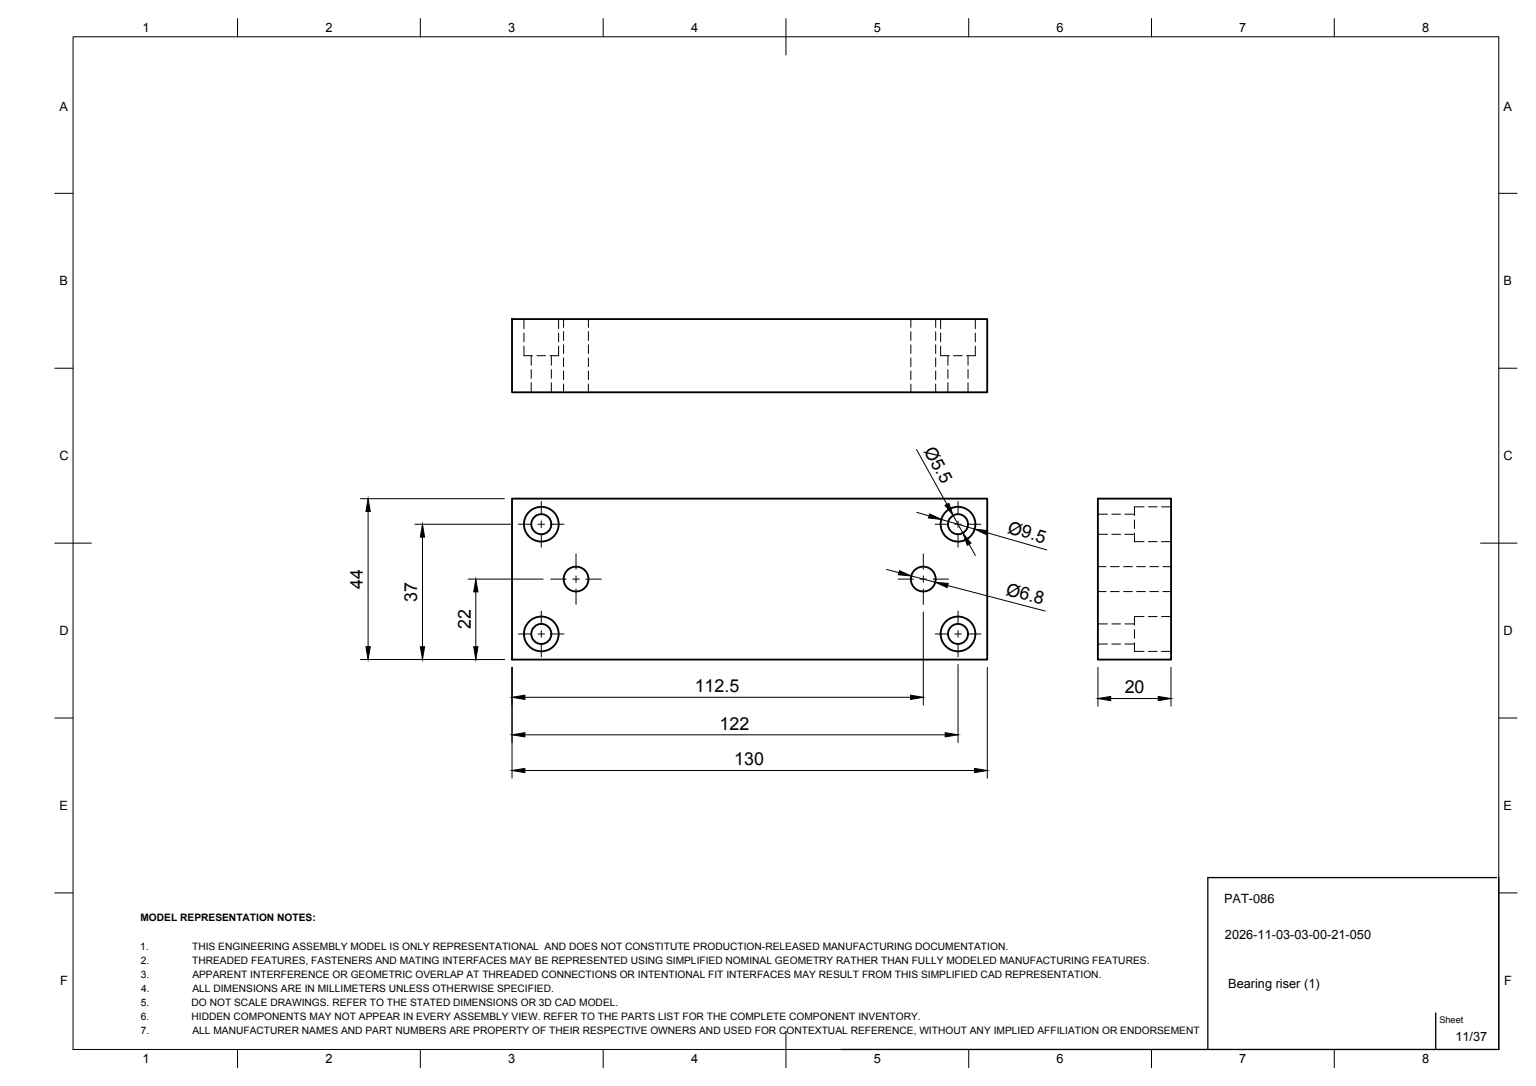
ISO-10303-21;
HEADER;
/* Generated by software containing ST-Developer
 * from STEP Tools, Inc. (www.steptools.com) 
 */

FILE_DESCRIPTION(
/* description */ ('Ratchet and pawl hand winch drum'),
/* implementation_level */ '2;1');

FILE_NAME(
/* name */ 'Bearing riser (1).step',
/* time_stamp */ '2026-10-27T12:42:58-07:00',
/* author */ (''),
/* organization */ (''),
/* preprocessor_version */ 'ST-DEVELOPER v20.2',
/* originating_system */ 'Autodesk Translation Framework v15.17.0.0',
/* authorisation */ '');

FILE_SCHEMA (('AUTOMOTIVE_DESIGN { 1 0 10303 214 3 1 1 }'));
ENDSEC;

DATA;
#10=MECHANICAL_DESIGN_GEOMETRIC_PRESENTATION_REPRESENTATION('',(#395),#11801);
#327=SHAPE_REPRESENTATION_RELATIONSHIP('SRR','None',#11953,#361);
#361=ADVANCED_BREP_SHAPE_REPRESENTATION('',(#430),#11770);
#395=STYLED_ITEM('',(#12213),#430);
#430=MANIFOLD_SOLID_BREP('Body1',#6272);
#496=FACE_BOUND('',#1294,.T.);
#497=FACE_BOUND('',#1297,.T.);
#498=FACE_BOUND('',#1302,.T.);
#499=FACE_BOUND('',#1305,.T.);
#500=FACE_BOUND('',#1315,.T.);
#501=FACE_BOUND('',#1316,.T.);
#502=FACE_BOUND('',#1317,.T.);
#503=FACE_BOUND('',#1318,.T.);
#504=FACE_BOUND('',#1319,.T.);
#505=FACE_BOUND('',#1320,.T.);
#506=FACE_BOUND('',#1322,.T.);
#507=FACE_BOUND('',#1323,.T.);
#508=FACE_BOUND('',#1324,.T.);
#509=FACE_BOUND('',#1325,.T.);
#510=FACE_BOUND('',#1326,.T.);
#511=FACE_BOUND('',#1327,.T.);
#633=PLANE('',#6795);
#634=PLANE('',#6800);
#635=PLANE('',#6809);
#636=PLANE('',#6814);
#637=PLANE('',#6826);
#638=PLANE('',#6827);
#639=PLANE('',#6828);
#640=PLANE('',#6829);
#641=PLANE('',#6830);
#642=PLANE('',#6831);
#896=FACE_OUTER_BOUND('',#1292,.T.);
#897=FACE_OUTER_BOUND('',#1293,.T.);
#898=FACE_OUTER_BOUND('',#1295,.T.);
#899=FACE_OUTER_BOUND('',#1296,.T.);
#900=FACE_OUTER_BOUND('',#1298,.T.);
#901=FACE_OUTER_BOUND('',#1299,.T.);
#902=FACE_OUTER_BOUND('',#1300,.T.);
#903=FACE_OUTER_BOUND('',#1301,.T.);
#904=FACE_OUTER_BOUND('',#1303,.T.);
#905=FACE_OUTER_BOUND('',#1304,.T.);
#906=FACE_OUTER_BOUND('',#1306,.T.);
#907=FACE_OUTER_BOUND('',#1307,.T.);
#908=FACE_OUTER_BOUND('',#1308,.T.);
#909=FACE_OUTER_BOUND('',#1309,.T.);
#910=FACE_OUTER_BOUND('',#1310,.T.);
#911=FACE_OUTER_BOUND('',#1311,.T.);
#912=FACE_OUTER_BOUND('',#1312,.T.);
#913=FACE_OUTER_BOUND('',#1313,.T.);
#914=FACE_OUTER_BOUND('',#1314,.T.);
#915=FACE_OUTER_BOUND('',#1321,.T.);
#1292=EDGE_LOOP('',(#4487,#4488,#4489,#4490));
#1293=EDGE_LOOP('',(#4491));
#1294=EDGE_LOOP('',(#4492));
#1295=EDGE_LOOP('',(#4493,#4494,#4495,#4496));
#1296=EDGE_LOOP('',(#4497));
#1297=EDGE_LOOP('',(#4498));
#1298=EDGE_LOOP('',(#4499,#4500,#4501,#4502));
#1299=EDGE_LOOP('',(#4503,#4504,#4505,#4506));
#1300=EDGE_LOOP('',(#4507,#4508,#4509,#4510));
#1301=EDGE_LOOP('',(#4511));
#1302=EDGE_LOOP('',(#4512));
#1303=EDGE_LOOP('',(#4513,#4514,#4515,#4516));
#1304=EDGE_LOOP('',(#4517));
#1305=EDGE_LOOP('',(#4518));
#1306=EDGE_LOOP('',(#4519,#4520,#4521,#4522));
#1307=EDGE_LOOP('',(#4523,#4524,#4525,#4526));
#1308=EDGE_LOOP('',(#4527,#4528,#4529,#4530));
#1309=EDGE_LOOP('',(#4531,#4532,#4533,#4534));
#1310=EDGE_LOOP('',(#4535,#4536,#4537,#4538));
#1311=EDGE_LOOP('',(#4539,#4540,#4541,#4542));
#1312=EDGE_LOOP('',(#4543,#4544,#4545,#4546));
#1313=EDGE_LOOP('',(#4547,#4548,#4549,#4550));
#1314=EDGE_LOOP('',(#4551,#4552,#4553,#4554));
#1315=EDGE_LOOP('',(#4555));
#1316=EDGE_LOOP('',(#4556));
#1317=EDGE_LOOP('',(#4557));
#1318=EDGE_LOOP('',(#4558));
#1319=EDGE_LOOP('',(#4559));
#1320=EDGE_LOOP('',(#4560));
#1321=EDGE_LOOP('',(#4561,#4562,#4563,#4564));
#1322=EDGE_LOOP('',(#4565));
#1323=EDGE_LOOP('',(#4566));
#1324=EDGE_LOOP('',(#4567));
#1325=EDGE_LOOP('',(#4568));
#1326=EDGE_LOOP('',(#4569));
#1327=EDGE_LOOP('',(#4570));
#1769=LINE('',#9496,#2280);
#1770=LINE('',#9505,#2281);
#1771=LINE('',#9513,#2282);
#1772=LINE('',#9517,#2283);
#1773=LINE('',#9522,#2284);
#1774=LINE('',#9531,#2285);
#1775=LINE('',#9539,#2286);
#1776=LINE('',#9543,#2287);
#1777=LINE('',#9548,#2288);
#1778=LINE('',#9554,#2289);
#1779=LINE('',#9559,#2290);
#1780=LINE('',#9561,#2291);
#1781=LINE('',#9563,#2292);
#1782=LINE('',#9564,#2293);
#1783=LINE('',#9567,#2294);
#1784=LINE('',#9569,#2295);
#1785=LINE('',#9570,#2296);
#1786=LINE('',#9573,#2297);
#1787=LINE('',#9575,#2298);
#1788=LINE('',#9576,#2299);
#1789=LINE('',#9578,#2300);
#1790=LINE('',#9579,#2301);
#2280=VECTOR('',#7660,0.475);
#2281=VECTOR('',#7671,0.475);
#2282=VECTOR('',#7682,0.275);
#2283=VECTOR('',#7687,0.275);
#2284=VECTOR('',#7692,0.475);
#2285=VECTOR('',#7703,0.475);
#2286=VECTOR('',#7714,0.275);
#2287=VECTOR('',#7719,0.275);
#2288=VECTOR('',#7724,0.34);
#2289=VECTOR('',#7731,0.34);
#2290=VECTOR('',#7736,1.);
#2291=VECTOR('',#7737,1.);
#2292=VECTOR('',#7738,1.);
#2293=VECTOR('',#7739,1.);
#2294=VECTOR('',#7742,1.);
#2295=VECTOR('',#7743,1.);
#2296=VECTOR('',#7744,1.);
#2297=VECTOR('',#7747,1.);
#2298=VECTOR('',#7748,1.);
#2299=VECTOR('',#7749,1.);
#2300=VECTOR('',#7752,1.);
#2301=VECTOR('',#7753,1.);
#2767=CIRCLE('',#6793,0.475);
#2768=CIRCLE('',#6794,0.475);
#2769=CIRCLE('',#6796,0.275);
#2770=CIRCLE('',#6798,0.475);
#2771=CIRCLE('',#6799,0.475);
#2772=CIRCLE('',#6801,0.275);
#2773=CIRCLE('',#6803,0.275);
#2774=CIRCLE('',#6805,0.275);
#2775=CIRCLE('',#6807,0.475);
#2776=CIRCLE('',#6808,0.475);
#2777=CIRCLE('',#6810,0.275);
#2778=CIRCLE('',#6812,0.475);
#2779=CIRCLE('',#6813,0.475);
#2780=CIRCLE('',#6815,0.275);
#2781=CIRCLE('',#6817,0.275);
#2782=CIRCLE('',#6819,0.275);
#2783=CIRCLE('',#6821,0.34);
#2784=CIRCLE('',#6822,0.34);
#2785=CIRCLE('',#6824,0.34);
#2786=CIRCLE('',#6825,0.34);
#3022=VERTEX_POINT('',#9493);
#3023=VERTEX_POINT('',#9495);
#3024=VERTEX_POINT('',#9499);
#3025=VERTEX_POINT('',#9502);
#3026=VERTEX_POINT('',#9504);
#3027=VERTEX_POINT('',#9508);
#3028=VERTEX_POINT('',#9511);
#3029=VERTEX_POINT('',#9515);
#3030=VERTEX_POINT('',#9519);
#3031=VERTEX_POINT('',#9521);
#3032=VERTEX_POINT('',#9525);
#3033=VERTEX_POINT('',#9528);
#3034=VERTEX_POINT('',#9530);
#3035=VERTEX_POINT('',#9534);
#3036=VERTEX_POINT('',#9537);
#3037=VERTEX_POINT('',#9541);
#3038=VERTEX_POINT('',#9545);
#3039=VERTEX_POINT('',#9547);
#3040=VERTEX_POINT('',#9551);
#3041=VERTEX_POINT('',#9553);
#3042=VERTEX_POINT('',#9557);
#3043=VERTEX_POINT('',#9558);
#3044=VERTEX_POINT('',#9560);
#3045=VERTEX_POINT('',#9562);
#3046=VERTEX_POINT('',#9566);
#3047=VERTEX_POINT('',#9568);
#3048=VERTEX_POINT('',#9572);
#3049=VERTEX_POINT('',#9574);
#3587=EDGE_CURVE('',#3022,#3022,#2767,.T.);
#3588=EDGE_CURVE('',#3022,#3023,#1769,.T.);
#3589=EDGE_CURVE('',#3023,#3023,#2768,.T.);
#3590=EDGE_CURVE('',#3024,#3024,#2769,.T.);
#3591=EDGE_CURVE('',#3025,#3025,#2770,.T.);
#3592=EDGE_CURVE('',#3025,#3026,#1770,.T.);
#3593=EDGE_CURVE('',#3026,#3026,#2771,.T.);
#3594=EDGE_CURVE('',#3027,#3027,#2772,.T.);
#3595=EDGE_CURVE('',#3028,#3028,#2773,.T.);
#3596=EDGE_CURVE('',#3028,#3024,#1771,.T.);
#3597=EDGE_CURVE('',#3029,#3029,#2774,.T.);
#3598=EDGE_CURVE('',#3029,#3027,#1772,.T.);
#3599=EDGE_CURVE('',#3030,#3030,#2775,.T.);
#3600=EDGE_CURVE('',#3030,#3031,#1773,.T.);
#3601=EDGE_CURVE('',#3031,#3031,#2776,.T.);
#3602=EDGE_CURVE('',#3032,#3032,#2777,.T.);
#3603=EDGE_CURVE('',#3033,#3033,#2778,.T.);
#3604=EDGE_CURVE('',#3033,#3034,#1774,.T.);
#3605=EDGE_CURVE('',#3034,#3034,#2779,.T.);
#3606=EDGE_CURVE('',#3035,#3035,#2780,.T.);
#3607=EDGE_CURVE('',#3036,#3036,#2781,.T.);
#3608=EDGE_CURVE('',#3036,#3032,#1775,.T.);
#3609=EDGE_CURVE('',#3037,#3037,#2782,.T.);
#3610=EDGE_CURVE('',#3037,#3035,#1776,.T.);
#3611=EDGE_CURVE('',#3038,#3038,#2783,.T.);
#3612=EDGE_CURVE('',#3038,#3039,#1777,.T.);
#3613=EDGE_CURVE('',#3039,#3039,#2784,.T.);
#3614=EDGE_CURVE('',#3040,#3040,#2785,.T.);
#3615=EDGE_CURVE('',#3040,#3041,#1778,.T.);
#3616=EDGE_CURVE('',#3041,#3041,#2786,.T.);
#3617=EDGE_CURVE('',#3042,#3043,#1779,.T.);
#3618=EDGE_CURVE('',#3043,#3044,#1780,.T.);
#3619=EDGE_CURVE('',#3045,#3044,#1781,.T.);
#3620=EDGE_CURVE('',#3042,#3045,#1782,.T.);
#3621=EDGE_CURVE('',#3046,#3042,#1783,.T.);
#3622=EDGE_CURVE('',#3047,#3045,#1784,.T.);
#3623=EDGE_CURVE('',#3046,#3047,#1785,.T.);
#3624=EDGE_CURVE('',#3048,#3046,#1786,.T.);
#3625=EDGE_CURVE('',#3049,#3047,#1787,.T.);
#3626=EDGE_CURVE('',#3048,#3049,#1788,.T.);
#3627=EDGE_CURVE('',#3043,#3048,#1789,.T.);
#3628=EDGE_CURVE('',#3044,#3049,#1790,.T.);
#4487=ORIENTED_EDGE('',*,*,#3587,.F.);
#4488=ORIENTED_EDGE('',*,*,#3588,.T.);
#4489=ORIENTED_EDGE('',*,*,#3589,.F.);
#4490=ORIENTED_EDGE('',*,*,#3588,.F.);
#4491=ORIENTED_EDGE('',*,*,#3587,.T.);
#4492=ORIENTED_EDGE('',*,*,#3590,.F.);
#4493=ORIENTED_EDGE('',*,*,#3591,.F.);
#4494=ORIENTED_EDGE('',*,*,#3592,.T.);
#4495=ORIENTED_EDGE('',*,*,#3593,.F.);
#4496=ORIENTED_EDGE('',*,*,#3592,.F.);
#4497=ORIENTED_EDGE('',*,*,#3591,.T.);
#4498=ORIENTED_EDGE('',*,*,#3594,.F.);
#4499=ORIENTED_EDGE('',*,*,#3595,.F.);
#4500=ORIENTED_EDGE('',*,*,#3596,.T.);
#4501=ORIENTED_EDGE('',*,*,#3590,.T.);
#4502=ORIENTED_EDGE('',*,*,#3596,.F.);
#4503=ORIENTED_EDGE('',*,*,#3597,.F.);
#4504=ORIENTED_EDGE('',*,*,#3598,.T.);
#4505=ORIENTED_EDGE('',*,*,#3594,.T.);
#4506=ORIENTED_EDGE('',*,*,#3598,.F.);
#4507=ORIENTED_EDGE('',*,*,#3599,.F.);
#4508=ORIENTED_EDGE('',*,*,#3600,.T.);
#4509=ORIENTED_EDGE('',*,*,#3601,.F.);
#4510=ORIENTED_EDGE('',*,*,#3600,.F.);
#4511=ORIENTED_EDGE('',*,*,#3599,.T.);
#4512=ORIENTED_EDGE('',*,*,#3602,.F.);
#4513=ORIENTED_EDGE('',*,*,#3603,.F.);
#4514=ORIENTED_EDGE('',*,*,#3604,.T.);
#4515=ORIENTED_EDGE('',*,*,#3605,.F.);
#4516=ORIENTED_EDGE('',*,*,#3604,.F.);
#4517=ORIENTED_EDGE('',*,*,#3603,.T.);
#4518=ORIENTED_EDGE('',*,*,#3606,.F.);
#4519=ORIENTED_EDGE('',*,*,#3607,.F.);
#4520=ORIENTED_EDGE('',*,*,#3608,.T.);
#4521=ORIENTED_EDGE('',*,*,#3602,.T.);
#4522=ORIENTED_EDGE('',*,*,#3608,.F.);
#4523=ORIENTED_EDGE('',*,*,#3609,.F.);
#4524=ORIENTED_EDGE('',*,*,#3610,.T.);
#4525=ORIENTED_EDGE('',*,*,#3606,.T.);
#4526=ORIENTED_EDGE('',*,*,#3610,.F.);
#4527=ORIENTED_EDGE('',*,*,#3611,.F.);
#4528=ORIENTED_EDGE('',*,*,#3612,.T.);
#4529=ORIENTED_EDGE('',*,*,#3613,.F.);
#4530=ORIENTED_EDGE('',*,*,#3612,.F.);
#4531=ORIENTED_EDGE('',*,*,#3614,.F.);
#4532=ORIENTED_EDGE('',*,*,#3615,.T.);
#4533=ORIENTED_EDGE('',*,*,#3616,.F.);
#4534=ORIENTED_EDGE('',*,*,#3615,.F.);
#4535=ORIENTED_EDGE('',*,*,#3617,.T.);
#4536=ORIENTED_EDGE('',*,*,#3618,.T.);
#4537=ORIENTED_EDGE('',*,*,#3619,.F.);
#4538=ORIENTED_EDGE('',*,*,#3620,.F.);
#4539=ORIENTED_EDGE('',*,*,#3621,.T.);
#4540=ORIENTED_EDGE('',*,*,#3620,.T.);
#4541=ORIENTED_EDGE('',*,*,#3622,.F.);
#4542=ORIENTED_EDGE('',*,*,#3623,.F.);
#4543=ORIENTED_EDGE('',*,*,#3624,.T.);
#4544=ORIENTED_EDGE('',*,*,#3623,.T.);
#4545=ORIENTED_EDGE('',*,*,#3625,.F.);
#4546=ORIENTED_EDGE('',*,*,#3626,.F.);
#4547=ORIENTED_EDGE('',*,*,#3627,.T.);
#4548=ORIENTED_EDGE('',*,*,#3626,.T.);
#4549=ORIENTED_EDGE('',*,*,#3628,.F.);
#4550=ORIENTED_EDGE('',*,*,#3618,.F.);
#4551=ORIENTED_EDGE('',*,*,#3628,.T.);
#4552=ORIENTED_EDGE('',*,*,#3625,.T.);
#4553=ORIENTED_EDGE('',*,*,#3622,.T.);
#4554=ORIENTED_EDGE('',*,*,#3619,.T.);
#4555=ORIENTED_EDGE('',*,*,#3616,.T.);
#4556=ORIENTED_EDGE('',*,*,#3613,.T.);
#4557=ORIENTED_EDGE('',*,*,#3605,.T.);
#4558=ORIENTED_EDGE('',*,*,#3601,.T.);
#4559=ORIENTED_EDGE('',*,*,#3593,.T.);
#4560=ORIENTED_EDGE('',*,*,#3589,.T.);
#4561=ORIENTED_EDGE('',*,*,#3627,.F.);
#4562=ORIENTED_EDGE('',*,*,#3617,.F.);
#4563=ORIENTED_EDGE('',*,*,#3621,.F.);
#4564=ORIENTED_EDGE('',*,*,#3624,.F.);
#4565=ORIENTED_EDGE('',*,*,#3595,.T.);
#4566=ORIENTED_EDGE('',*,*,#3597,.T.);
#4567=ORIENTED_EDGE('',*,*,#3607,.T.);
#4568=ORIENTED_EDGE('',*,*,#3609,.T.);
#4569=ORIENTED_EDGE('',*,*,#3611,.T.);
#4570=ORIENTED_EDGE('',*,*,#3614,.T.);
#5831=CYLINDRICAL_SURFACE('',#6792,0.475);
#5832=CYLINDRICAL_SURFACE('',#6797,0.475);
#5833=CYLINDRICAL_SURFACE('',#6802,0.275);
#5834=CYLINDRICAL_SURFACE('',#6804,0.275);
#5835=CYLINDRICAL_SURFACE('',#6806,0.475);
#5836=CYLINDRICAL_SURFACE('',#6811,0.475);
#5837=CYLINDRICAL_SURFACE('',#6816,0.275);
#5838=CYLINDRICAL_SURFACE('',#6818,0.275);
#5839=CYLINDRICAL_SURFACE('',#6820,0.34);
#5840=CYLINDRICAL_SURFACE('',#6823,0.34);
#5966=ADVANCED_FACE('',(#896),#5831,.F.);
#5967=ADVANCED_FACE('',(#897,#496),#633,.T.);
#5968=ADVANCED_FACE('',(#898),#5832,.F.);
#5969=ADVANCED_FACE('',(#899,#497),#634,.T.);
#5970=ADVANCED_FACE('',(#900),#5833,.F.);
#5971=ADVANCED_FACE('',(#901),#5834,.F.);
#5972=ADVANCED_FACE('',(#902),#5835,.F.);
#5973=ADVANCED_FACE('',(#903,#498),#635,.T.);
#5974=ADVANCED_FACE('',(#904),#5836,.F.);
#5975=ADVANCED_FACE('',(#905,#499),#636,.T.);
#5976=ADVANCED_FACE('',(#906),#5837,.F.);
#5977=ADVANCED_FACE('',(#907),#5838,.F.);
#5978=ADVANCED_FACE('',(#908),#5839,.F.);
#5979=ADVANCED_FACE('',(#909),#5840,.F.);
#5980=ADVANCED_FACE('',(#910),#637,.T.);
#5981=ADVANCED_FACE('',(#911),#638,.T.);
#5982=ADVANCED_FACE('',(#912),#639,.T.);
#5983=ADVANCED_FACE('',(#913),#640,.T.);
#5984=ADVANCED_FACE('',(#914,#500,#501,#502,#503,#504,#505),#641,.T.);
#5985=ADVANCED_FACE('',(#915,#506,#507,#508,#509,#510,#511),#642,.F.);
#6272=CLOSED_SHELL('',(#5966,#5967,#5968,#5969,#5970,#5971,#5972,#5973,
#5974,#5975,#5976,#5977,#5978,#5979,#5980,#5981,#5982,#5983,#5984,#5985));
#6791=AXIS2_PLACEMENT_3D('',#9491,#7654,#7655);
#6792=AXIS2_PLACEMENT_3D('',#9492,#7656,#7657);
#6793=AXIS2_PLACEMENT_3D('',#9494,#7658,#7659);
#6794=AXIS2_PLACEMENT_3D('',#9497,#7661,#7662);
#6795=AXIS2_PLACEMENT_3D('',#9498,#7663,#7664);
#6796=AXIS2_PLACEMENT_3D('',#9500,#7665,#7666);
#6797=AXIS2_PLACEMENT_3D('',#9501,#7667,#7668);
#6798=AXIS2_PLACEMENT_3D('',#9503,#7669,#7670);
#6799=AXIS2_PLACEMENT_3D('',#9506,#7672,#7673);
#6800=AXIS2_PLACEMENT_3D('',#9507,#7674,#7675);
#6801=AXIS2_PLACEMENT_3D('',#9509,#7676,#7677);
#6802=AXIS2_PLACEMENT_3D('',#9510,#7678,#7679);
#6803=AXIS2_PLACEMENT_3D('',#9512,#7680,#7681);
#6804=AXIS2_PLACEMENT_3D('',#9514,#7683,#7684);
#6805=AXIS2_PLACEMENT_3D('',#9516,#7685,#7686);
#6806=AXIS2_PLACEMENT_3D('',#9518,#7688,#7689);
#6807=AXIS2_PLACEMENT_3D('',#9520,#7690,#7691);
#6808=AXIS2_PLACEMENT_3D('',#9523,#7693,#7694);
#6809=AXIS2_PLACEMENT_3D('',#9524,#7695,#7696);
#6810=AXIS2_PLACEMENT_3D('',#9526,#7697,#7698);
#6811=AXIS2_PLACEMENT_3D('',#9527,#7699,#7700);
#6812=AXIS2_PLACEMENT_3D('',#9529,#7701,#7702);
#6813=AXIS2_PLACEMENT_3D('',#9532,#7704,#7705);
#6814=AXIS2_PLACEMENT_3D('',#9533,#7706,#7707);
#6815=AXIS2_PLACEMENT_3D('',#9535,#7708,#7709);
#6816=AXIS2_PLACEMENT_3D('',#9536,#7710,#7711);
#6817=AXIS2_PLACEMENT_3D('',#9538,#7712,#7713);
#6818=AXIS2_PLACEMENT_3D('',#9540,#7715,#7716);
#6819=AXIS2_PLACEMENT_3D('',#9542,#7717,#7718);
#6820=AXIS2_PLACEMENT_3D('',#9544,#7720,#7721);
#6821=AXIS2_PLACEMENT_3D('',#9546,#7722,#7723);
#6822=AXIS2_PLACEMENT_3D('',#9549,#7725,#7726);
#6823=AXIS2_PLACEMENT_3D('',#9550,#7727,#7728);
#6824=AXIS2_PLACEMENT_3D('',#9552,#7729,#7730);
#6825=AXIS2_PLACEMENT_3D('',#9555,#7732,#7733);
#6826=AXIS2_PLACEMENT_3D('',#9556,#7734,#7735);
#6827=AXIS2_PLACEMENT_3D('',#9565,#7740,#7741);
#6828=AXIS2_PLACEMENT_3D('',#9571,#7745,#7746);
#6829=AXIS2_PLACEMENT_3D('',#9577,#7750,#7751);
#6830=AXIS2_PLACEMENT_3D('',#9580,#7754,#7755);
#6831=AXIS2_PLACEMENT_3D('',#9581,#7756,#7757);
#7654=DIRECTION('axis',(0.,0.,1.));
#7655=DIRECTION('refdir',(1.,0.,0.));
#7656=DIRECTION('center_axis',(0.,0.,1.));
#7657=DIRECTION('ref_axis',(1.,0.,0.));
#7658=DIRECTION('center_axis',(0.,0.,1.));
#7659=DIRECTION('ref_axis',(1.,0.,0.));
#7660=DIRECTION('',(0.,0.,1.));
#7661=DIRECTION('center_axis',(0.,0.,-1.));
#7662=DIRECTION('ref_axis',(1.,0.,0.));
#7663=DIRECTION('center_axis',(0.,0.,1.));
#7664=DIRECTION('ref_axis',(1.,0.,0.));
#7665=DIRECTION('center_axis',(0.,0.,1.));
#7666=DIRECTION('ref_axis',(1.,0.,0.));
#7667=DIRECTION('center_axis',(0.,0.,1.));
#7668=DIRECTION('ref_axis',(1.,0.,0.));
#7669=DIRECTION('center_axis',(0.,0.,1.));
#7670=DIRECTION('ref_axis',(1.,0.,0.));
#7671=DIRECTION('',(0.,0.,1.));
#7672=DIRECTION('center_axis',(0.,0.,-1.));
#7673=DIRECTION('ref_axis',(1.,0.,0.));
#7674=DIRECTION('center_axis',(0.,0.,1.));
#7675=DIRECTION('ref_axis',(1.,0.,0.));
#7676=DIRECTION('center_axis',(0.,0.,1.));
#7677=DIRECTION('ref_axis',(1.,0.,0.));
#7678=DIRECTION('center_axis',(0.,0.,1.));
#7679=DIRECTION('ref_axis',(1.,0.,0.));
#7680=DIRECTION('center_axis',(0.,0.,1.));
#7681=DIRECTION('ref_axis',(1.,0.,0.));
#7682=DIRECTION('',(0.,0.,1.));
#7683=DIRECTION('center_axis',(0.,0.,1.));
#7684=DIRECTION('ref_axis',(1.,0.,0.));
#7685=DIRECTION('center_axis',(0.,0.,1.));
#7686=DIRECTION('ref_axis',(1.,0.,0.));
#7687=DIRECTION('',(0.,0.,1.));
#7688=DIRECTION('center_axis',(0.,0.,1.));
#7689=DIRECTION('ref_axis',(1.,0.,0.));
#7690=DIRECTION('center_axis',(0.,0.,1.));
#7691=DIRECTION('ref_axis',(1.,0.,0.));
#7692=DIRECTION('',(0.,0.,1.));
#7693=DIRECTION('center_axis',(0.,0.,-1.));
#7694=DIRECTION('ref_axis',(1.,0.,0.));
#7695=DIRECTION('center_axis',(0.,0.,1.));
#7696=DIRECTION('ref_axis',(1.,0.,0.));
#7697=DIRECTION('center_axis',(0.,0.,1.));
#7698=DIRECTION('ref_axis',(1.,0.,0.));
#7699=DIRECTION('center_axis',(0.,0.,1.));
#7700=DIRECTION('ref_axis',(1.,0.,0.));
#7701=DIRECTION('center_axis',(0.,0.,1.));
#7702=DIRECTION('ref_axis',(1.,0.,0.));
#7703=DIRECTION('',(0.,0.,1.));
#7704=DIRECTION('center_axis',(0.,0.,-1.));
#7705=DIRECTION('ref_axis',(1.,0.,0.));
#7706=DIRECTION('center_axis',(0.,0.,1.));
#7707=DIRECTION('ref_axis',(1.,0.,0.));
#7708=DIRECTION('center_axis',(0.,0.,1.));
#7709=DIRECTION('ref_axis',(1.,0.,0.));
#7710=DIRECTION('center_axis',(0.,0.,1.));
#7711=DIRECTION('ref_axis',(1.,0.,0.));
#7712=DIRECTION('center_axis',(0.,0.,1.));
#7713=DIRECTION('ref_axis',(1.,0.,0.));
#7714=DIRECTION('',(0.,0.,1.));
#7715=DIRECTION('center_axis',(0.,0.,1.));
#7716=DIRECTION('ref_axis',(1.,0.,0.));
#7717=DIRECTION('center_axis',(0.,0.,1.));
#7718=DIRECTION('ref_axis',(1.,0.,0.));
#7719=DIRECTION('',(0.,0.,1.));
#7720=DIRECTION('center_axis',(0.,0.,1.));
#7721=DIRECTION('ref_axis',(1.,0.,0.));
#7722=DIRECTION('center_axis',(0.,0.,1.));
#7723=DIRECTION('ref_axis',(1.,0.,0.));
#7724=DIRECTION('',(0.,0.,1.));
#7725=DIRECTION('center_axis',(0.,0.,-1.));
#7726=DIRECTION('ref_axis',(1.,0.,0.));
#7727=DIRECTION('center_axis',(0.,0.,1.));
#7728=DIRECTION('ref_axis',(1.,0.,0.));
#7729=DIRECTION('center_axis',(0.,0.,1.));
#7730=DIRECTION('ref_axis',(1.,0.,0.));
#7731=DIRECTION('',(0.,0.,1.));
#7732=DIRECTION('center_axis',(0.,0.,-1.));
#7733=DIRECTION('ref_axis',(1.,0.,0.));
#7734=DIRECTION('center_axis',(0.,1.,0.));
#7735=DIRECTION('ref_axis',(-1.,0.,0.));
#7736=DIRECTION('',(-1.,0.,0.));
#7737=DIRECTION('',(0.,0.,1.));
#7738=DIRECTION('',(-1.,0.,0.));
#7739=DIRECTION('',(0.,0.,1.));
#7740=DIRECTION('center_axis',(1.,0.,0.));
#7741=DIRECTION('ref_axis',(0.,1.,0.));
#7742=DIRECTION('',(0.,1.,0.));
#7743=DIRECTION('',(0.,1.,0.));
#7744=DIRECTION('',(0.,0.,1.));
#7745=DIRECTION('center_axis',(0.,-1.,0.));
#7746=DIRECTION('ref_axis',(1.,0.,0.));
#7747=DIRECTION('',(1.,0.,0.));
#7748=DIRECTION('',(1.,0.,0.));
#7749=DIRECTION('',(0.,0.,1.));
#7750=DIRECTION('center_axis',(-1.,0.,0.));
#7751=DIRECTION('ref_axis',(0.,-1.,0.));
#7752=DIRECTION('',(0.,-1.,0.));
#7753=DIRECTION('',(0.,-1.,0.));
#7754=DIRECTION('center_axis',(0.,0.,1.));
#7755=DIRECTION('ref_axis',(1.,0.,0.));
#7756=DIRECTION('center_axis',(0.,0.,1.));
#7757=DIRECTION('ref_axis',(1.,0.,0.));
#9491=CARTESIAN_POINT('',(0.,0.,0.));
#9492=CARTESIAN_POINT('Origin',(5.7,14.5,2.2));
#9493=CARTESIAN_POINT('',(5.225,14.5,2.2));
#9494=CARTESIAN_POINT('Origin',(5.7,14.5,2.2));
#9495=CARTESIAN_POINT('',(5.225,14.5,3.2));
#9496=CARTESIAN_POINT('',(5.225,14.5,2.2));
#9497=CARTESIAN_POINT('Origin',(5.7,14.5,3.2));
#9498=CARTESIAN_POINT('Origin',(5.7,14.5,2.2));
#9499=CARTESIAN_POINT('',(5.425,14.5,2.2));
#9500=CARTESIAN_POINT('Origin',(5.7,14.5,2.2));
#9501=CARTESIAN_POINT('Origin',(5.7,17.5,2.2));
#9502=CARTESIAN_POINT('',(5.225,17.5,2.2));
#9503=CARTESIAN_POINT('Origin',(5.7,17.5,2.2));
#9504=CARTESIAN_POINT('',(5.225,17.5,3.2));
#9505=CARTESIAN_POINT('',(5.225,17.5,2.2));
#9506=CARTESIAN_POINT('Origin',(5.7,17.5,3.2));
#9507=CARTESIAN_POINT('Origin',(5.7,17.5,2.2));
#9508=CARTESIAN_POINT('',(5.425,17.5,2.2));
#9509=CARTESIAN_POINT('Origin',(5.7,17.5,2.2));
#9510=CARTESIAN_POINT('Origin',(5.7,14.5,1.1));
#9511=CARTESIAN_POINT('',(5.425,14.5,1.2));
#9512=CARTESIAN_POINT('Origin',(5.7,14.5,1.2));
#9513=CARTESIAN_POINT('',(5.425,14.5,1.1));
#9514=CARTESIAN_POINT('Origin',(5.7,17.5,1.1));
#9515=CARTESIAN_POINT('',(5.425,17.5,1.2));
#9516=CARTESIAN_POINT('Origin',(5.7,17.5,1.2));
#9517=CARTESIAN_POINT('',(5.425,17.5,1.1));
#9518=CARTESIAN_POINT('Origin',(-5.7,14.5,2.2));
#9519=CARTESIAN_POINT('',(-6.175,14.5,2.2));
#9520=CARTESIAN_POINT('Origin',(-5.7,14.5,2.2));
#9521=CARTESIAN_POINT('',(-6.175,14.5,3.2));
#9522=CARTESIAN_POINT('',(-6.175,14.5,2.2));
#9523=CARTESIAN_POINT('Origin',(-5.7,14.5,3.2));
#9524=CARTESIAN_POINT('Origin',(-5.7,14.5,2.2));
#9525=CARTESIAN_POINT('',(-5.975,14.5,2.2));
#9526=CARTESIAN_POINT('Origin',(-5.7,14.5,2.2));
#9527=CARTESIAN_POINT('Origin',(-5.7,17.5,2.2));
#9528=CARTESIAN_POINT('',(-6.175,17.5,2.2));
#9529=CARTESIAN_POINT('Origin',(-5.7,17.5,2.2));
#9530=CARTESIAN_POINT('',(-6.175,17.5,3.2));
#9531=CARTESIAN_POINT('',(-6.175,17.5,2.2));
#9532=CARTESIAN_POINT('Origin',(-5.7,17.5,3.2));
#9533=CARTESIAN_POINT('Origin',(-5.7,17.5,2.2));
#9534=CARTESIAN_POINT('',(-5.975,17.5,2.2));
#9535=CARTESIAN_POINT('Origin',(-5.7,17.5,2.2));
#9536=CARTESIAN_POINT('Origin',(-5.7,14.5,1.1));
#9537=CARTESIAN_POINT('',(-5.975,14.5,1.2));
#9538=CARTESIAN_POINT('Origin',(-5.7,14.5,1.2));
#9539=CARTESIAN_POINT('',(-5.975,14.5,1.1));
#9540=CARTESIAN_POINT('Origin',(-5.7,17.5,1.1));
#9541=CARTESIAN_POINT('',(-5.975,17.5,1.2));
#9542=CARTESIAN_POINT('Origin',(-5.7,17.5,1.2));
#9543=CARTESIAN_POINT('',(-5.975,17.5,1.1));
#9544=CARTESIAN_POINT('Origin',(-4.75,16.,1.1));
#9545=CARTESIAN_POINT('',(-5.09,16.,1.2));
#9546=CARTESIAN_POINT('Origin',(-4.75,16.,1.2));
#9547=CARTESIAN_POINT('',(-5.09,16.,3.2));
#9548=CARTESIAN_POINT('',(-5.09,16.,1.1));
#9549=CARTESIAN_POINT('Origin',(-4.75,16.,3.2));
#9550=CARTESIAN_POINT('Origin',(4.75,16.,1.1));
#9551=CARTESIAN_POINT('',(4.41,16.,1.2));
#9552=CARTESIAN_POINT('Origin',(4.75,16.,1.2));
#9553=CARTESIAN_POINT('',(4.41,16.,3.2));
#9554=CARTESIAN_POINT('',(4.41,16.,1.1));
#9555=CARTESIAN_POINT('Origin',(4.75,16.,3.2));
#9556=CARTESIAN_POINT('Origin',(6.5,18.2,1.2));
#9557=CARTESIAN_POINT('',(6.5,18.2,1.2));
#9558=CARTESIAN_POINT('',(-6.5,18.2,1.2));
#9559=CARTESIAN_POINT('',(6.5,18.2,1.2));
#9560=CARTESIAN_POINT('',(-6.5,18.2,3.2));
#9561=CARTESIAN_POINT('',(-6.5,18.2,1.2));
#9562=CARTESIAN_POINT('',(6.5,18.2,3.2));
#9563=CARTESIAN_POINT('',(6.5,18.2,3.2));
#9564=CARTESIAN_POINT('',(6.5,18.2,1.2));
#9565=CARTESIAN_POINT('Origin',(6.5,13.8,1.2));
#9566=CARTESIAN_POINT('',(6.5,13.8,1.2));
#9567=CARTESIAN_POINT('',(6.5,13.8,1.2));
#9568=CARTESIAN_POINT('',(6.5,13.8,3.2));
#9569=CARTESIAN_POINT('',(6.5,13.8,3.2));
#9570=CARTESIAN_POINT('',(6.5,13.8,1.2));
#9571=CARTESIAN_POINT('Origin',(-6.5,13.8,1.2));
#9572=CARTESIAN_POINT('',(-6.5,13.8,1.2));
#9573=CARTESIAN_POINT('',(-6.5,13.8,1.2));
#9574=CARTESIAN_POINT('',(-6.5,13.8,3.2));
#9575=CARTESIAN_POINT('',(-6.5,13.8,3.2));
#9576=CARTESIAN_POINT('',(-6.5,13.8,1.2));
#9577=CARTESIAN_POINT('Origin',(-6.5,18.2,1.2));
#9578=CARTESIAN_POINT('',(-6.5,18.2,1.2));
#9579=CARTESIAN_POINT('',(-6.5,18.2,3.2));
#9580=CARTESIAN_POINT('Origin',(0.,16.,3.2));
#9581=CARTESIAN_POINT('Origin',(0.,16.,1.2));
#11730=UNCERTAINTY_MEASURE_WITH_UNIT(LENGTH_MEASURE(0.001),#11802,
'DISTANCE_ACCURACY_VALUE',
'Maximum model space distance between geometric entities at asserted c
onnectivities');
#11761=UNCERTAINTY_MEASURE_WITH_UNIT(LENGTH_MEASURE(0.001),#11802,
'DISTANCE_ACCURACY_VALUE',
'Maximum model space distance between geometric entities at asserted c
onnectivities');
#11770=(
GEOMETRIC_REPRESENTATION_CONTEXT(3)
GLOBAL_UNCERTAINTY_ASSIGNED_CONTEXT((#11730))
GLOBAL_UNIT_ASSIGNED_CONTEXT((#11802,#11804,#11805))
REPRESENTATION_CONTEXT('','3D')
);
#11801=(
GEOMETRIC_REPRESENTATION_CONTEXT(3)
GLOBAL_UNCERTAINTY_ASSIGNED_CONTEXT((#11761))
GLOBAL_UNIT_ASSIGNED_CONTEXT((#11802,#11804,#11805))
REPRESENTATION_CONTEXT('','3D')
);
#11802=(
LENGTH_UNIT()
NAMED_UNIT(*)
SI_UNIT(.CENTI.,.METRE.)
);
#11804=(
NAMED_UNIT(*)
PLANE_ANGLE_UNIT()
SI_UNIT($,.RADIAN.)
);
#11805=(
NAMED_UNIT(*)
SI_UNIT($,.STERADIAN.)
SOLID_ANGLE_UNIT()
);
#11814=SHAPE_DEFINITION_REPRESENTATION(#11853,#11953);
#11853=PRODUCT_DEFINITION_SHAPE('',$,#11993);
#11953=SHAPE_REPRESENTATION('',(#6791),#11770);
#11984=PRODUCT_DEFINITION_CONTEXT('part definition',#12103,'design');
#11993=PRODUCT_DEFINITION('Bearing riser (1)','Bearing riser (1)',#12032,
#11984);
#12032=PRODUCT_DEFINITION_FORMATION('',$,#12113);
#12103=APPLICATION_CONTEXT(
'Core Data for Automotive Mechanical Design Process');
#12104=PRODUCT_CONTEXT('part definition',#12103,'mechanical');
#12113=PRODUCT('Bearing riser (1)','Bearing riser (1)','Bearing riser (1)',(#12104));
#12207=COLOUR_RGB('Grey',0.48,0.52,0.57);
#12208=FILL_AREA_STYLE_COLOUR('',#12207);
#12209=FILL_AREA_STYLE('',(#12208));
#12210=SURFACE_STYLE_FILL_AREA(#12209);
#12211=SURFACE_SIDE_STYLE('',(#12210));
#12212=SURFACE_STYLE_USAGE(.BOTH.,#12211);
#12213=PRESENTATION_STYLE_ASSIGNMENT((#12212));
ENDSEC;
END-ISO-10303-21;
